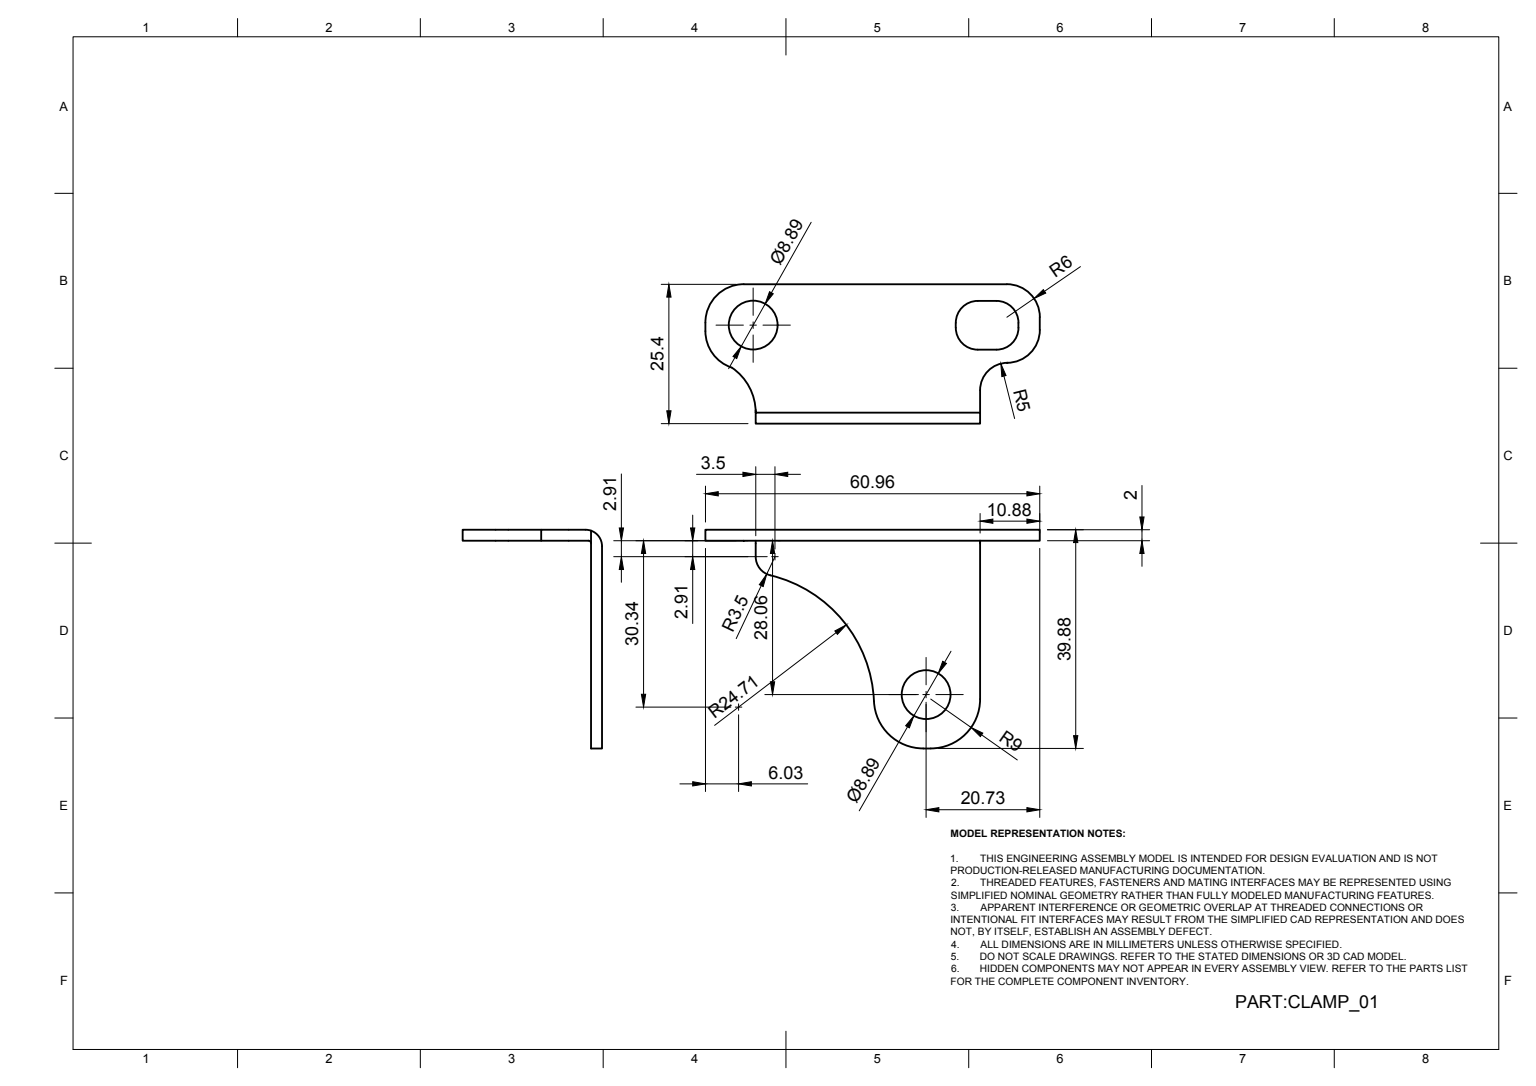
ISO-10303-21;
HEADER;
/* Generated by software containing ST-Developer
 * from STEP Tools, Inc. (www.steptools.com) 
 */

FILE_DESCRIPTION(
/* description */ (''),
/* implementation_level */ '2;1');

FILE_NAME(
/* name */ 'Clamp_01.step',
/* time_stamp */ '2026-10-04T16:49:01-07:00',
/* author */ (''),
/* organization */ (''),
/* preprocessor_version */ 'ST-DEVELOPER v20.2',
/* originating_system */ 'Autodesk Translation Framework v15.15.0.0',
/* authorisation */ '');

FILE_SCHEMA (('AUTOMOTIVE_DESIGN { 1 0 10303 214 3 1 1 }'));
ENDSEC;

DATA;
#10=MECHANICAL_DESIGN_GEOMETRIC_PRESENTATION_REPRESENTATION('',(#80),#51553);
#64=SHAPE_REPRESENTATION_RELATIONSHIP('SRR','None',#51585,#72);
#72=ADVANCED_BREP_SHAPE_REPRESENTATION('',(#89),#51545);
#80=STYLED_ITEM('',(#51634),#89);
#89=MANIFOLD_SOLID_BREP('Body1',#4259);
#98=FACE_BOUND('',#379,.T.);
#99=FACE_BOUND('',#382,.T.);
#100=FACE_BOUND('',#411,.T.);
#101=FACE_BOUND('',#412,.T.);
#102=FACE_BOUND('',#414,.T.);
#103=FACE_BOUND('',#415,.T.);
#120=PLANE('',#4363);
#121=PLANE('',#4365);
#122=PLANE('',#4371);
#123=PLANE('',#4372);
#124=PLANE('',#4383);
#125=PLANE('',#4386);
#126=PLANE('',#4390);
#127=PLANE('',#4394);
#128=PLANE('',#4398);
#129=PLANE('',#4402);
#130=PLANE('',#4415);
#131=PLANE('',#4419);
#132=PLANE('',#4423);
#133=PLANE('',#4427);
#134=PLANE('',#4428);
#135=PLANE('',#4429);
#181=FACE_OUTER_BOUND('',#376,.T.);
#182=FACE_OUTER_BOUND('',#377,.T.);
#183=FACE_OUTER_BOUND('',#378,.T.);
#184=FACE_OUTER_BOUND('',#380,.T.);
#185=FACE_OUTER_BOUND('',#381,.T.);
#186=FACE_OUTER_BOUND('',#383,.T.);
#187=FACE_OUTER_BOUND('',#384,.T.);
#188=FACE_OUTER_BOUND('',#385,.T.);
#189=FACE_OUTER_BOUND('',#386,.T.);
#190=FACE_OUTER_BOUND('',#387,.T.);
#191=FACE_OUTER_BOUND('',#388,.T.);
#192=FACE_OUTER_BOUND('',#389,.T.);
#193=FACE_OUTER_BOUND('',#390,.T.);
#194=FACE_OUTER_BOUND('',#391,.T.);
#195=FACE_OUTER_BOUND('',#392,.T.);
#196=FACE_OUTER_BOUND('',#393,.T.);
#197=FACE_OUTER_BOUND('',#394,.T.);
#198=FACE_OUTER_BOUND('',#395,.T.);
#199=FACE_OUTER_BOUND('',#396,.T.);
#200=FACE_OUTER_BOUND('',#397,.T.);
#201=FACE_OUTER_BOUND('',#398,.T.);
#202=FACE_OUTER_BOUND('',#399,.T.);
#203=FACE_OUTER_BOUND('',#400,.T.);
#204=FACE_OUTER_BOUND('',#401,.T.);
#205=FACE_OUTER_BOUND('',#402,.T.);
#206=FACE_OUTER_BOUND('',#403,.T.);
#207=FACE_OUTER_BOUND('',#404,.T.);
#208=FACE_OUTER_BOUND('',#405,.T.);
#209=FACE_OUTER_BOUND('',#406,.T.);
#210=FACE_OUTER_BOUND('',#407,.T.);
#211=FACE_OUTER_BOUND('',#408,.T.);
#212=FACE_OUTER_BOUND('',#409,.T.);
#213=FACE_OUTER_BOUND('',#410,.T.);
#214=FACE_OUTER_BOUND('',#413,.T.);
#376=EDGE_LOOP('',(#2629,#2630,#2631,#2632,#2633,#2634,#2635));
#377=EDGE_LOOP('',(#2636,#2637,#2638,#2639,#2640,#2641));
#378=EDGE_LOOP('',(#2642,#2643,#2644,#2645,#2646,#2647,#2648,#2649,#2650,
#2651));
#379=EDGE_LOOP('',(#2652));
#380=EDGE_LOOP('',(#2653,#2654,#2655,#2656));
#381=EDGE_LOOP('',(#2657,#2658,#2659,#2660,#2661,#2662,#2663,#2664));
#382=EDGE_LOOP('',(#2665));
#383=EDGE_LOOP('',(#2666,#2667,#2668,#2669));
#384=EDGE_LOOP('',(#2670,#2671,#2672,#2673));
#385=EDGE_LOOP('',(#2674,#2675,#2676,#2677));
#386=EDGE_LOOP('',(#2678,#2679,#2680,#2681));
#387=EDGE_LOOP('',(#2682,#2683,#2684,#2685));
#388=EDGE_LOOP('',(#2686,#2687,#2688,#2689));
#389=EDGE_LOOP('',(#2690,#2691,#2692,#2693));
#390=EDGE_LOOP('',(#2694,#2695,#2696,#2697,#2698,#2699,#2700));
#391=EDGE_LOOP('',(#2701,#2702,#2703,#2704));
#392=EDGE_LOOP('',(#2705,#2706,#2707,#2708));
#393=EDGE_LOOP('',(#2709,#2710,#2711,#2712));
#394=EDGE_LOOP('',(#2713,#2714,#2715,#2716));
#395=EDGE_LOOP('',(#2717,#2718,#2719,#2720));
#396=EDGE_LOOP('',(#2721,#2722,#2723,#2724));
#397=EDGE_LOOP('',(#2725,#2726,#2727,#2728));
#398=EDGE_LOOP('',(#2729,#2730,#2731,#2732));
#399=EDGE_LOOP('',(#2733,#2734,#2735,#2736));
#400=EDGE_LOOP('',(#2737,#2738,#2739,#2740));
#401=EDGE_LOOP('',(#2741,#2742,#2743,#2744,#2745));
#402=EDGE_LOOP('',(#2746,#2747,#2748,#2749));
#403=EDGE_LOOP('',(#2750,#2751,#2752,#2753));
#404=EDGE_LOOP('',(#2754,#2755,#2756,#2757));
#405=EDGE_LOOP('',(#2758,#2759,#2760,#2761));
#406=EDGE_LOOP('',(#2762,#2763,#2764,#2765));
#407=EDGE_LOOP('',(#2766,#2767,#2768,#2769));
#408=EDGE_LOOP('',(#2770,#2771,#2772,#2773));
#409=EDGE_LOOP('',(#2774,#2775,#2776,#2777));
#410=EDGE_LOOP('',(#2778,#2779,#2780,#2781,#2782,#2783,#2784,#2785,#2786,
#2787,#2788,#2789,#2790));
#411=EDGE_LOOP('',(#2791,#2792,#2793,#2794,#2795,#2796,#2797,#2798));
#412=EDGE_LOOP('',(#2799));
#413=EDGE_LOOP('',(#2800,#2801,#2802,#2803,#2804,#2805,#2806,#2807,#2808,
#2809,#2810,#2811));
#414=EDGE_LOOP('',(#2812,#2813,#2814,#2815,#2816,#2817,#2818,#2819));
#415=EDGE_LOOP('',(#2820));
#593=CIRCLE('',#4360,3.);
#594=CIRCLE('',#4361,3.);
#595=CIRCLE('',#4362,3.);
#596=CIRCLE('',#4364,0.5);
#597=CIRCLE('',#4366,3.5);
#598=CIRCLE('',#4367,24.7141941620437);
#599=CIRCLE('',#4368,9.);
#600=CIRCLE('',#4369,9.);
#601=CIRCLE('',#4370,4.445);
#602=CIRCLE('',#4373,9.);
#603=CIRCLE('',#4374,9.);
#604=CIRCLE('',#4375,24.7141941620437);
#605=CIRCLE('',#4376,3.5);
#606=CIRCLE('',#4377,4.445);
#607=CIRCLE('',#4379,0.5);
#608=CIRCLE('',#4388,4.445);
#609=CIRCLE('',#4389,4.445);
#610=CIRCLE('',#4392,3.99999999999999);
#611=CIRCLE('',#4393,3.99999999999999);
#612=CIRCLE('',#4396,4.00000000000001);
#613=CIRCLE('',#4397,4.00000000000001);
#614=CIRCLE('',#4400,4.00000000000001);
#615=CIRCLE('',#4401,4.00000000000001);
#616=CIRCLE('',#4404,4.00000000000001);
#617=CIRCLE('',#4405,4.00000000000001);
#618=CIRCLE('',#4407,6.99999999999999);
#619=CIRCLE('',#4408,6.99999999999999);
#620=CIRCLE('',#4410,9.9094315895918);
#621=CIRCLE('',#4411,9.9094315895918);
#622=CIRCLE('',#4413,5.);
#623=CIRCLE('',#4414,5.);
#624=CIRCLE('',#4417,5.99999999999999);
#625=CIRCLE('',#4418,5.99999999999999);
#626=CIRCLE('',#4421,5.99999999999999);
#627=CIRCLE('',#4422,5.99999999999999);
#628=CIRCLE('',#4425,7.);
#629=CIRCLE('',#4426,7.);
#711=LINE('',#5537,#939);
#712=LINE('',#5541,#940);
#713=LINE('',#5545,#941);
#714=LINE('',#5549,#942);
#715=LINE('',#5551,#943);
#716=LINE('',#5553,#944);
#717=LINE('',#5556,#945);
#718=LINE('',#5559,#946);
#719=LINE('',#5561,#947);
#720=LINE('',#5569,#948);
#721=LINE('',#5572,#949);
#722=LINE('',#5577,#950);
#723=LINE('',#5578,#951);
#724=LINE('',#5583,#952);
#725=LINE('',#5590,#953);
#726=LINE('',#5596,#954);
#727=LINE('',#5598,#955);
#728=LINE('',#5599,#956);
#729=LINE('',#5601,#957);
#730=LINE('',#5603,#958);
#731=LINE('',#5605,#959);
#732=LINE('',#5608,#960);
#733=LINE('',#5611,#961);
#734=LINE('',#5612,#962);
#735=LINE('',#5617,#963);
#736=LINE('',#5622,#964);
#737=LINE('',#5624,#965);
#738=LINE('',#5626,#966);
#739=LINE('',#5627,#967);
#740=LINE('',#5632,#968);
#741=LINE('',#5636,#969);
#742=LINE('',#5638,#970);
#743=LINE('',#5639,#971);
#744=LINE('',#5644,#972);
#745=LINE('',#5648,#973);
#746=LINE('',#5650,#974);
#747=LINE('',#5651,#975);
#748=LINE('',#5656,#976);
#749=LINE('',#5660,#977);
#750=LINE('',#5662,#978);
#751=LINE('',#5663,#979);
#752=LINE('',#5672,#980);
#753=LINE('',#5675,#981);
#754=LINE('',#5683,#982);
#755=LINE('',#5687,#983);
#756=LINE('',#5689,#984);
#757=LINE('',#5690,#985);
#758=LINE('',#5695,#986);
#759=LINE('',#5699,#987);
#760=LINE('',#5701,#988);
#761=LINE('',#5702,#989);
#762=LINE('',#5707,#990);
#763=LINE('',#5711,#991);
#764=LINE('',#5713,#992);
#765=LINE('',#5714,#993);
#766=LINE('',#5719,#994);
#767=LINE('',#5722,#995);
#768=LINE('',#5723,#996);
#939=VECTOR('',#4677,10.);
#940=VECTOR('',#4680,10.);
#941=VECTOR('',#4683,10.);
#942=VECTOR('',#4688,10.);
#943=VECTOR('',#4689,10.);
#944=VECTOR('',#4690,10.);
#945=VECTOR('',#4693,10.);
#946=VECTOR('',#4696,10.);
#947=VECTOR('',#4697,10.);
#948=VECTOR('',#4704,10.);
#949=VECTOR('',#4707,10.);
#950=VECTOR('',#4712,10.);
#951=VECTOR('',#4713,10.);
#952=VECTOR('',#4718,10.);
#953=VECTOR('',#4725,10.);
#954=VECTOR('',#4732,10.);
#955=VECTOR('',#4735,10.);
#956=VECTOR('',#4736,10.);
#957=VECTOR('',#4739,9.);
#958=VECTOR('',#4742,10.);
#959=VECTOR('',#4745,9.);
#960=VECTOR('',#4750,4.445);
#961=VECTOR('',#4753,10.);
#962=VECTOR('',#4754,10.);
#963=VECTOR('',#4759,4.445);
#964=VECTOR('',#4764,10.);
#965=VECTOR('',#4765,10.);
#966=VECTOR('',#4766,10.);
#967=VECTOR('',#4767,10.);
#968=VECTOR('',#4772,10.);
#969=VECTOR('',#4777,10.);
#970=VECTOR('',#4778,10.);
#971=VECTOR('',#4779,10.);
#972=VECTOR('',#4784,10.);
#973=VECTOR('',#4789,10.);
#974=VECTOR('',#4790,10.);
#975=VECTOR('',#4791,10.);
#976=VECTOR('',#4796,10.);
#977=VECTOR('',#4801,10.);
#978=VECTOR('',#4802,10.);
#979=VECTOR('',#4803,10.);
#980=VECTOR('',#4814,10.);
#981=VECTOR('',#4817,10.);
#982=VECTOR('',#4828,10.);
#983=VECTOR('',#4833,10.);
#984=VECTOR('',#4834,10.);
#985=VECTOR('',#4835,10.);
#986=VECTOR('',#4840,10.);
#987=VECTOR('',#4845,10.);
#988=VECTOR('',#4846,10.);
#989=VECTOR('',#4847,10.);
#990=VECTOR('',#4852,10.);
#991=VECTOR('',#4857,10.);
#992=VECTOR('',#4858,10.);
#993=VECTOR('',#4859,10.);
#994=VECTOR('',#4864,10.);
#995=VECTOR('',#4869,10.);
#996=VECTOR('',#4870,10.);
#1167=B_SPLINE_CURVE_WITH_KNOTS('',3,(#5532,#5533,#5534,#5535),
 .UNSPECIFIED.,.F.,.F.,(4,4),(0.459706916456031,0.558076312618392),
 .UNSPECIFIED.);
#1482=VERTEX_POINT('',#5530);
#1483=VERTEX_POINT('',#5531);
#1484=VERTEX_POINT('',#5536);
#1485=VERTEX_POINT('',#5538);
#1486=VERTEX_POINT('',#5540);
#1487=VERTEX_POINT('',#5542);
#1488=VERTEX_POINT('',#5544);
#1489=VERTEX_POINT('',#5548);
#1490=VERTEX_POINT('',#5550);
#1491=VERTEX_POINT('',#5552);
#1492=VERTEX_POINT('',#5554);
#1493=VERTEX_POINT('',#5558);
#1494=VERTEX_POINT('',#5560);
#1495=VERTEX_POINT('',#5562);
#1496=VERTEX_POINT('',#5564);
#1497=VERTEX_POINT('',#5566);
#1498=VERTEX_POINT('',#5568);
#1499=VERTEX_POINT('',#5570);
#1500=VERTEX_POINT('',#5573);
#1501=VERTEX_POINT('',#5576);
#1502=VERTEX_POINT('',#5580);
#1503=VERTEX_POINT('',#5582);
#1504=VERTEX_POINT('',#5584);
#1505=VERTEX_POINT('',#5586);
#1506=VERTEX_POINT('',#5588);
#1507=VERTEX_POINT('',#5591);
#1508=VERTEX_POINT('',#5594);
#1509=VERTEX_POINT('',#5610);
#1510=VERTEX_POINT('',#5614);
#1511=VERTEX_POINT('',#5616);
#1512=VERTEX_POINT('',#5620);
#1513=VERTEX_POINT('',#5621);
#1514=VERTEX_POINT('',#5623);
#1515=VERTEX_POINT('',#5625);
#1516=VERTEX_POINT('',#5629);
#1517=VERTEX_POINT('',#5631);
#1518=VERTEX_POINT('',#5635);
#1519=VERTEX_POINT('',#5637);
#1520=VERTEX_POINT('',#5641);
#1521=VERTEX_POINT('',#5643);
#1522=VERTEX_POINT('',#5647);
#1523=VERTEX_POINT('',#5649);
#1524=VERTEX_POINT('',#5653);
#1525=VERTEX_POINT('',#5655);
#1526=VERTEX_POINT('',#5659);
#1527=VERTEX_POINT('',#5661);
#1528=VERTEX_POINT('',#5668);
#1529=VERTEX_POINT('',#5669);
#1530=VERTEX_POINT('',#5671);
#1531=VERTEX_POINT('',#5673);
#1532=VERTEX_POINT('',#5680);
#1533=VERTEX_POINT('',#5682);
#1534=VERTEX_POINT('',#5686);
#1535=VERTEX_POINT('',#5688);
#1536=VERTEX_POINT('',#5692);
#1537=VERTEX_POINT('',#5694);
#1538=VERTEX_POINT('',#5698);
#1539=VERTEX_POINT('',#5700);
#1540=VERTEX_POINT('',#5704);
#1541=VERTEX_POINT('',#5706);
#1542=VERTEX_POINT('',#5710);
#1543=VERTEX_POINT('',#5712);
#1544=VERTEX_POINT('',#5716);
#1545=VERTEX_POINT('',#5718);
#1968=EDGE_CURVE('',#1482,#1483,#1167,.T.);
#1969=EDGE_CURVE('',#1484,#1482,#711,.T.);
#1970=EDGE_CURVE('',#1485,#1484,#593,.T.);
#1971=EDGE_CURVE('',#1486,#1485,#712,.T.);
#1972=EDGE_CURVE('',#1487,#1486,#594,.T.);
#1973=EDGE_CURVE('',#1488,#1487,#713,.T.);
#1974=EDGE_CURVE('',#1483,#1488,#595,.T.);
#1975=EDGE_CURVE('',#1489,#1484,#714,.T.);
#1976=EDGE_CURVE('',#1489,#1490,#715,.T.);
#1977=EDGE_CURVE('',#1490,#1491,#716,.T.);
#1978=EDGE_CURVE('',#1491,#1492,#596,.T.);
#1979=EDGE_CURVE('',#1485,#1492,#717,.T.);
#1980=EDGE_CURVE('',#1492,#1493,#718,.T.);
#1981=EDGE_CURVE('',#1493,#1494,#719,.T.);
#1982=EDGE_CURVE('',#1494,#1495,#597,.T.);
#1983=EDGE_CURVE('',#1496,#1495,#598,.T.);
#1984=EDGE_CURVE('',#1496,#1497,#599,.T.);
#1985=EDGE_CURVE('',#1497,#1498,#720,.T.);
#1986=EDGE_CURVE('',#1498,#1499,#600,.T.);
#1987=EDGE_CURVE('',#1486,#1499,#721,.F.);
#1988=EDGE_CURVE('',#1500,#1500,#601,.T.);
#1989=EDGE_CURVE('',#1499,#1501,#722,.T.);
#1990=EDGE_CURVE('',#1487,#1501,#723,.T.);
#1991=EDGE_CURVE('',#1501,#1502,#602,.T.);
#1992=EDGE_CURVE('',#1502,#1503,#724,.T.);
#1993=EDGE_CURVE('',#1503,#1504,#603,.T.);
#1994=EDGE_CURVE('',#1505,#1504,#604,.T.);
#1995=EDGE_CURVE('',#1505,#1506,#605,.T.);
#1996=EDGE_CURVE('',#1488,#1506,#725,.F.);
#1997=EDGE_CURVE('',#1507,#1507,#606,.T.);
#1998=EDGE_CURVE('',#1508,#1493,#607,.F.);
#1999=EDGE_CURVE('',#1508,#1491,#726,.T.);
#2000=EDGE_CURVE('',#1495,#1505,#727,.T.);
#2001=EDGE_CURVE('',#1506,#1494,#728,.T.);
#2002=EDGE_CURVE('',#1504,#1496,#729,.T.);
#2003=EDGE_CURVE('',#1502,#1498,#730,.T.);
#2004=EDGE_CURVE('',#1497,#1503,#731,.T.);
#2005=EDGE_CURVE('',#1507,#1500,#732,.T.);
#2006=EDGE_CURVE('',#1508,#1509,#733,.T.);
#2007=EDGE_CURVE('',#1483,#1509,#734,.T.);
#2008=EDGE_CURVE('',#1510,#1510,#608,.T.);
#2009=EDGE_CURVE('',#1510,#1511,#735,.T.);
#2010=EDGE_CURVE('',#1511,#1511,#609,.T.);
#2011=EDGE_CURVE('',#1512,#1513,#736,.T.);
#2012=EDGE_CURVE('',#1512,#1514,#737,.T.);
#2013=EDGE_CURVE('',#1514,#1515,#738,.T.);
#2014=EDGE_CURVE('',#1513,#1515,#739,.T.);
#2015=EDGE_CURVE('',#1516,#1512,#610,.T.);
#2016=EDGE_CURVE('',#1516,#1517,#740,.T.);
#2017=EDGE_CURVE('',#1517,#1514,#611,.T.);
#2018=EDGE_CURVE('',#1518,#1516,#741,.T.);
#2019=EDGE_CURVE('',#1518,#1519,#742,.T.);
#2020=EDGE_CURVE('',#1519,#1517,#743,.T.);
#2021=EDGE_CURVE('',#1520,#1518,#612,.T.);
#2022=EDGE_CURVE('',#1520,#1521,#744,.T.);
#2023=EDGE_CURVE('',#1521,#1519,#613,.T.);
#2024=EDGE_CURVE('',#1522,#1520,#745,.T.);
#2025=EDGE_CURVE('',#1522,#1523,#746,.T.);
#2026=EDGE_CURVE('',#1523,#1521,#747,.T.);
#2027=EDGE_CURVE('',#1524,#1522,#614,.T.);
#2028=EDGE_CURVE('',#1524,#1525,#748,.T.);
#2029=EDGE_CURVE('',#1525,#1523,#615,.T.);
#2030=EDGE_CURVE('',#1526,#1524,#749,.T.);
#2031=EDGE_CURVE('',#1526,#1527,#750,.T.);
#2032=EDGE_CURVE('',#1527,#1525,#751,.T.);
#2033=EDGE_CURVE('',#1513,#1526,#616,.T.);
#2034=EDGE_CURVE('',#1515,#1527,#617,.T.);
#2035=EDGE_CURVE('',#1528,#1529,#618,.T.);
#2036=EDGE_CURVE('',#1528,#1530,#752,.T.);
#2037=EDGE_CURVE('',#1530,#1531,#619,.T.);
#2038=EDGE_CURVE('',#1529,#1531,#753,.T.);
#2039=EDGE_CURVE('',#1509,#1530,#620,.T.);
#2040=EDGE_CURVE('',#1528,#1482,#621,.T.);
#2041=EDGE_CURVE('',#1489,#1532,#622,.T.);
#2042=EDGE_CURVE('',#1532,#1533,#754,.T.);
#2043=EDGE_CURVE('',#1533,#1490,#623,.T.);
#2044=EDGE_CURVE('',#1534,#1532,#755,.T.);
#2045=EDGE_CURVE('',#1534,#1535,#756,.T.);
#2046=EDGE_CURVE('',#1535,#1533,#757,.T.);
#2047=EDGE_CURVE('',#1536,#1534,#624,.T.);
#2048=EDGE_CURVE('',#1536,#1537,#758,.T.);
#2049=EDGE_CURVE('',#1537,#1535,#625,.T.);
#2050=EDGE_CURVE('',#1538,#1536,#759,.T.);
#2051=EDGE_CURVE('',#1538,#1539,#760,.T.);
#2052=EDGE_CURVE('',#1539,#1537,#761,.T.);
#2053=EDGE_CURVE('',#1540,#1538,#626,.T.);
#2054=EDGE_CURVE('',#1540,#1541,#762,.T.);
#2055=EDGE_CURVE('',#1541,#1539,#627,.T.);
#2056=EDGE_CURVE('',#1542,#1540,#763,.T.);
#2057=EDGE_CURVE('',#1542,#1543,#764,.T.);
#2058=EDGE_CURVE('',#1543,#1541,#765,.T.);
#2059=EDGE_CURVE('',#1544,#1542,#628,.T.);
#2060=EDGE_CURVE('',#1544,#1545,#766,.T.);
#2061=EDGE_CURVE('',#1545,#1543,#629,.T.);
#2062=EDGE_CURVE('',#1529,#1544,#767,.T.);
#2063=EDGE_CURVE('',#1531,#1545,#768,.T.);
#2629=ORIENTED_EDGE('',*,*,#1968,.F.);
#2630=ORIENTED_EDGE('',*,*,#1969,.F.);
#2631=ORIENTED_EDGE('',*,*,#1970,.F.);
#2632=ORIENTED_EDGE('',*,*,#1971,.F.);
#2633=ORIENTED_EDGE('',*,*,#1972,.F.);
#2634=ORIENTED_EDGE('',*,*,#1973,.F.);
#2635=ORIENTED_EDGE('',*,*,#1974,.F.);
#2636=ORIENTED_EDGE('',*,*,#1970,.T.);
#2637=ORIENTED_EDGE('',*,*,#1975,.F.);
#2638=ORIENTED_EDGE('',*,*,#1976,.T.);
#2639=ORIENTED_EDGE('',*,*,#1977,.T.);
#2640=ORIENTED_EDGE('',*,*,#1978,.T.);
#2641=ORIENTED_EDGE('',*,*,#1979,.F.);
#2642=ORIENTED_EDGE('',*,*,#1971,.T.);
#2643=ORIENTED_EDGE('',*,*,#1979,.T.);
#2644=ORIENTED_EDGE('',*,*,#1980,.T.);
#2645=ORIENTED_EDGE('',*,*,#1981,.T.);
#2646=ORIENTED_EDGE('',*,*,#1982,.T.);
#2647=ORIENTED_EDGE('',*,*,#1983,.F.);
#2648=ORIENTED_EDGE('',*,*,#1984,.T.);
#2649=ORIENTED_EDGE('',*,*,#1985,.T.);
#2650=ORIENTED_EDGE('',*,*,#1986,.T.);
#2651=ORIENTED_EDGE('',*,*,#1987,.F.);
#2652=ORIENTED_EDGE('',*,*,#1988,.F.);
#2653=ORIENTED_EDGE('',*,*,#1972,.T.);
#2654=ORIENTED_EDGE('',*,*,#1987,.T.);
#2655=ORIENTED_EDGE('',*,*,#1989,.T.);
#2656=ORIENTED_EDGE('',*,*,#1990,.F.);
#2657=ORIENTED_EDGE('',*,*,#1973,.T.);
#2658=ORIENTED_EDGE('',*,*,#1990,.T.);
#2659=ORIENTED_EDGE('',*,*,#1991,.T.);
#2660=ORIENTED_EDGE('',*,*,#1992,.T.);
#2661=ORIENTED_EDGE('',*,*,#1993,.T.);
#2662=ORIENTED_EDGE('',*,*,#1994,.F.);
#2663=ORIENTED_EDGE('',*,*,#1995,.T.);
#2664=ORIENTED_EDGE('',*,*,#1996,.F.);
#2665=ORIENTED_EDGE('',*,*,#1997,.F.);
#2666=ORIENTED_EDGE('',*,*,#1998,.T.);
#2667=ORIENTED_EDGE('',*,*,#1980,.F.);
#2668=ORIENTED_EDGE('',*,*,#1978,.F.);
#2669=ORIENTED_EDGE('',*,*,#1999,.F.);
#2670=ORIENTED_EDGE('',*,*,#1995,.F.);
#2671=ORIENTED_EDGE('',*,*,#2000,.F.);
#2672=ORIENTED_EDGE('',*,*,#1982,.F.);
#2673=ORIENTED_EDGE('',*,*,#2001,.F.);
#2674=ORIENTED_EDGE('',*,*,#2000,.T.);
#2675=ORIENTED_EDGE('',*,*,#1994,.T.);
#2676=ORIENTED_EDGE('',*,*,#2002,.T.);
#2677=ORIENTED_EDGE('',*,*,#1983,.T.);
#2678=ORIENTED_EDGE('',*,*,#1991,.F.);
#2679=ORIENTED_EDGE('',*,*,#1989,.F.);
#2680=ORIENTED_EDGE('',*,*,#1986,.F.);
#2681=ORIENTED_EDGE('',*,*,#2003,.F.);
#2682=ORIENTED_EDGE('',*,*,#2003,.T.);
#2683=ORIENTED_EDGE('',*,*,#1985,.F.);
#2684=ORIENTED_EDGE('',*,*,#2004,.T.);
#2685=ORIENTED_EDGE('',*,*,#1992,.F.);
#2686=ORIENTED_EDGE('',*,*,#1993,.F.);
#2687=ORIENTED_EDGE('',*,*,#2004,.F.);
#2688=ORIENTED_EDGE('',*,*,#1984,.F.);
#2689=ORIENTED_EDGE('',*,*,#2002,.F.);
#2690=ORIENTED_EDGE('',*,*,#1997,.T.);
#2691=ORIENTED_EDGE('',*,*,#2005,.T.);
#2692=ORIENTED_EDGE('',*,*,#1988,.T.);
#2693=ORIENTED_EDGE('',*,*,#2005,.F.);
#2694=ORIENTED_EDGE('',*,*,#1974,.T.);
#2695=ORIENTED_EDGE('',*,*,#1996,.T.);
#2696=ORIENTED_EDGE('',*,*,#2001,.T.);
#2697=ORIENTED_EDGE('',*,*,#1981,.F.);
#2698=ORIENTED_EDGE('',*,*,#1998,.F.);
#2699=ORIENTED_EDGE('',*,*,#2006,.T.);
#2700=ORIENTED_EDGE('',*,*,#2007,.F.);
#2701=ORIENTED_EDGE('',*,*,#2008,.T.);
#2702=ORIENTED_EDGE('',*,*,#2009,.T.);
#2703=ORIENTED_EDGE('',*,*,#2010,.F.);
#2704=ORIENTED_EDGE('',*,*,#2009,.F.);
#2705=ORIENTED_EDGE('',*,*,#2011,.F.);
#2706=ORIENTED_EDGE('',*,*,#2012,.T.);
#2707=ORIENTED_EDGE('',*,*,#2013,.T.);
#2708=ORIENTED_EDGE('',*,*,#2014,.F.);
#2709=ORIENTED_EDGE('',*,*,#2015,.F.);
#2710=ORIENTED_EDGE('',*,*,#2016,.T.);
#2711=ORIENTED_EDGE('',*,*,#2017,.T.);
#2712=ORIENTED_EDGE('',*,*,#2012,.F.);
#2713=ORIENTED_EDGE('',*,*,#2018,.F.);
#2714=ORIENTED_EDGE('',*,*,#2019,.T.);
#2715=ORIENTED_EDGE('',*,*,#2020,.T.);
#2716=ORIENTED_EDGE('',*,*,#2016,.F.);
#2717=ORIENTED_EDGE('',*,*,#2021,.F.);
#2718=ORIENTED_EDGE('',*,*,#2022,.T.);
#2719=ORIENTED_EDGE('',*,*,#2023,.T.);
#2720=ORIENTED_EDGE('',*,*,#2019,.F.);
#2721=ORIENTED_EDGE('',*,*,#2024,.F.);
#2722=ORIENTED_EDGE('',*,*,#2025,.T.);
#2723=ORIENTED_EDGE('',*,*,#2026,.T.);
#2724=ORIENTED_EDGE('',*,*,#2022,.F.);
#2725=ORIENTED_EDGE('',*,*,#2027,.F.);
#2726=ORIENTED_EDGE('',*,*,#2028,.T.);
#2727=ORIENTED_EDGE('',*,*,#2029,.T.);
#2728=ORIENTED_EDGE('',*,*,#2025,.F.);
#2729=ORIENTED_EDGE('',*,*,#2030,.F.);
#2730=ORIENTED_EDGE('',*,*,#2031,.T.);
#2731=ORIENTED_EDGE('',*,*,#2032,.T.);
#2732=ORIENTED_EDGE('',*,*,#2028,.F.);
#2733=ORIENTED_EDGE('',*,*,#2033,.F.);
#2734=ORIENTED_EDGE('',*,*,#2014,.T.);
#2735=ORIENTED_EDGE('',*,*,#2034,.T.);
#2736=ORIENTED_EDGE('',*,*,#2031,.F.);
#2737=ORIENTED_EDGE('',*,*,#2035,.F.);
#2738=ORIENTED_EDGE('',*,*,#2036,.T.);
#2739=ORIENTED_EDGE('',*,*,#2037,.T.);
#2740=ORIENTED_EDGE('',*,*,#2038,.F.);
#2741=ORIENTED_EDGE('',*,*,#1968,.T.);
#2742=ORIENTED_EDGE('',*,*,#2007,.T.);
#2743=ORIENTED_EDGE('',*,*,#2039,.T.);
#2744=ORIENTED_EDGE('',*,*,#2036,.F.);
#2745=ORIENTED_EDGE('',*,*,#2040,.T.);
#2746=ORIENTED_EDGE('',*,*,#2041,.T.);
#2747=ORIENTED_EDGE('',*,*,#2042,.T.);
#2748=ORIENTED_EDGE('',*,*,#2043,.T.);
#2749=ORIENTED_EDGE('',*,*,#1976,.F.);
#2750=ORIENTED_EDGE('',*,*,#2044,.F.);
#2751=ORIENTED_EDGE('',*,*,#2045,.T.);
#2752=ORIENTED_EDGE('',*,*,#2046,.T.);
#2753=ORIENTED_EDGE('',*,*,#2042,.F.);
#2754=ORIENTED_EDGE('',*,*,#2047,.F.);
#2755=ORIENTED_EDGE('',*,*,#2048,.T.);
#2756=ORIENTED_EDGE('',*,*,#2049,.T.);
#2757=ORIENTED_EDGE('',*,*,#2045,.F.);
#2758=ORIENTED_EDGE('',*,*,#2050,.F.);
#2759=ORIENTED_EDGE('',*,*,#2051,.T.);
#2760=ORIENTED_EDGE('',*,*,#2052,.T.);
#2761=ORIENTED_EDGE('',*,*,#2048,.F.);
#2762=ORIENTED_EDGE('',*,*,#2053,.F.);
#2763=ORIENTED_EDGE('',*,*,#2054,.T.);
#2764=ORIENTED_EDGE('',*,*,#2055,.T.);
#2765=ORIENTED_EDGE('',*,*,#2051,.F.);
#2766=ORIENTED_EDGE('',*,*,#2056,.F.);
#2767=ORIENTED_EDGE('',*,*,#2057,.T.);
#2768=ORIENTED_EDGE('',*,*,#2058,.T.);
#2769=ORIENTED_EDGE('',*,*,#2054,.F.);
#2770=ORIENTED_EDGE('',*,*,#2059,.F.);
#2771=ORIENTED_EDGE('',*,*,#2060,.T.);
#2772=ORIENTED_EDGE('',*,*,#2061,.T.);
#2773=ORIENTED_EDGE('',*,*,#2057,.F.);
#2774=ORIENTED_EDGE('',*,*,#2062,.F.);
#2775=ORIENTED_EDGE('',*,*,#2038,.T.);
#2776=ORIENTED_EDGE('',*,*,#2063,.T.);
#2777=ORIENTED_EDGE('',*,*,#2060,.F.);
#2778=ORIENTED_EDGE('',*,*,#2006,.F.);
#2779=ORIENTED_EDGE('',*,*,#1999,.T.);
#2780=ORIENTED_EDGE('',*,*,#1977,.F.);
#2781=ORIENTED_EDGE('',*,*,#2043,.F.);
#2782=ORIENTED_EDGE('',*,*,#2046,.F.);
#2783=ORIENTED_EDGE('',*,*,#2049,.F.);
#2784=ORIENTED_EDGE('',*,*,#2052,.F.);
#2785=ORIENTED_EDGE('',*,*,#2055,.F.);
#2786=ORIENTED_EDGE('',*,*,#2058,.F.);
#2787=ORIENTED_EDGE('',*,*,#2061,.F.);
#2788=ORIENTED_EDGE('',*,*,#2063,.F.);
#2789=ORIENTED_EDGE('',*,*,#2037,.F.);
#2790=ORIENTED_EDGE('',*,*,#2039,.F.);
#2791=ORIENTED_EDGE('',*,*,#2034,.F.);
#2792=ORIENTED_EDGE('',*,*,#2013,.F.);
#2793=ORIENTED_EDGE('',*,*,#2017,.F.);
#2794=ORIENTED_EDGE('',*,*,#2020,.F.);
#2795=ORIENTED_EDGE('',*,*,#2023,.F.);
#2796=ORIENTED_EDGE('',*,*,#2026,.F.);
#2797=ORIENTED_EDGE('',*,*,#2029,.F.);
#2798=ORIENTED_EDGE('',*,*,#2032,.F.);
#2799=ORIENTED_EDGE('',*,*,#2008,.F.);
#2800=ORIENTED_EDGE('',*,*,#1969,.T.);
#2801=ORIENTED_EDGE('',*,*,#2040,.F.);
#2802=ORIENTED_EDGE('',*,*,#2035,.T.);
#2803=ORIENTED_EDGE('',*,*,#2062,.T.);
#2804=ORIENTED_EDGE('',*,*,#2059,.T.);
#2805=ORIENTED_EDGE('',*,*,#2056,.T.);
#2806=ORIENTED_EDGE('',*,*,#2053,.T.);
#2807=ORIENTED_EDGE('',*,*,#2050,.T.);
#2808=ORIENTED_EDGE('',*,*,#2047,.T.);
#2809=ORIENTED_EDGE('',*,*,#2044,.T.);
#2810=ORIENTED_EDGE('',*,*,#2041,.F.);
#2811=ORIENTED_EDGE('',*,*,#1975,.T.);
#2812=ORIENTED_EDGE('',*,*,#2033,.T.);
#2813=ORIENTED_EDGE('',*,*,#2030,.T.);
#2814=ORIENTED_EDGE('',*,*,#2027,.T.);
#2815=ORIENTED_EDGE('',*,*,#2024,.T.);
#2816=ORIENTED_EDGE('',*,*,#2021,.T.);
#2817=ORIENTED_EDGE('',*,*,#2018,.T.);
#2818=ORIENTED_EDGE('',*,*,#2015,.T.);
#2819=ORIENTED_EDGE('',*,*,#2011,.T.);
#2820=ORIENTED_EDGE('',*,*,#2010,.T.);
#3951=CYLINDRICAL_SURFACE('',#4359,3.);
#3952=CYLINDRICAL_SURFACE('',#4378,0.5);
#3953=CYLINDRICAL_SURFACE('',#4380,3.5);
#3954=CYLINDRICAL_SURFACE('',#4381,24.7141941620437);
#3955=CYLINDRICAL_SURFACE('',#4382,9.);
#3956=CYLINDRICAL_SURFACE('',#4384,9.);
#3957=CYLINDRICAL_SURFACE('',#4385,4.445);
#3958=CYLINDRICAL_SURFACE('',#4387,4.445);
#3959=CYLINDRICAL_SURFACE('',#4391,3.99999999999999);
#3960=CYLINDRICAL_SURFACE('',#4395,4.00000000000001);
#3961=CYLINDRICAL_SURFACE('',#4399,4.00000000000001);
#3962=CYLINDRICAL_SURFACE('',#4403,4.00000000000001);
#3963=CYLINDRICAL_SURFACE('',#4406,6.99999999999999);
#3964=CYLINDRICAL_SURFACE('',#4409,9.9094315895918);
#3965=CYLINDRICAL_SURFACE('',#4412,5.);
#3966=CYLINDRICAL_SURFACE('',#4416,5.99999999999999);
#3967=CYLINDRICAL_SURFACE('',#4420,5.99999999999999);
#3968=CYLINDRICAL_SURFACE('',#4424,7.);
#4064=ADVANCED_FACE('',(#181),#3951,.T.);
#4065=ADVANCED_FACE('',(#182),#120,.F.);
#4066=ADVANCED_FACE('',(#183,#98),#121,.F.);
#4067=ADVANCED_FACE('',(#184),#122,.F.);
#4068=ADVANCED_FACE('',(#185,#99),#123,.F.);
#4069=ADVANCED_FACE('',(#186),#3952,.F.);
#4070=ADVANCED_FACE('',(#187),#3953,.T.);
#4071=ADVANCED_FACE('',(#188),#3954,.F.);
#4072=ADVANCED_FACE('',(#189),#3955,.T.);
#4073=ADVANCED_FACE('',(#190),#124,.F.);
#4074=ADVANCED_FACE('',(#191),#3956,.T.);
#4075=ADVANCED_FACE('',(#192),#3957,.F.);
#4076=ADVANCED_FACE('',(#193),#125,.F.);
#4077=ADVANCED_FACE('',(#194),#3958,.F.);
#4078=ADVANCED_FACE('',(#195),#126,.F.);
#4079=ADVANCED_FACE('',(#196),#3959,.F.);
#4080=ADVANCED_FACE('',(#197),#127,.F.);
#4081=ADVANCED_FACE('',(#198),#3960,.F.);
#4082=ADVANCED_FACE('',(#199),#128,.F.);
#4083=ADVANCED_FACE('',(#200),#3961,.F.);
#4084=ADVANCED_FACE('',(#201),#129,.F.);
#4085=ADVANCED_FACE('',(#202),#3962,.F.);
#4086=ADVANCED_FACE('',(#203),#3963,.T.);
#4087=ADVANCED_FACE('',(#204),#3964,.F.);
#4088=ADVANCED_FACE('',(#205),#3965,.F.);
#4089=ADVANCED_FACE('',(#206),#130,.F.);
#4090=ADVANCED_FACE('',(#207),#3966,.T.);
#4091=ADVANCED_FACE('',(#208),#131,.F.);
#4092=ADVANCED_FACE('',(#209),#3967,.T.);
#4093=ADVANCED_FACE('',(#210),#132,.F.);
#4094=ADVANCED_FACE('',(#211),#3968,.T.);
#4095=ADVANCED_FACE('',(#212),#133,.F.);
#4096=ADVANCED_FACE('',(#213,#100,#101),#134,.F.);
#4097=ADVANCED_FACE('',(#214,#102,#103),#135,.T.);
#4259=CLOSED_SHELL('',(#4064,#4065,#4066,#4067,#4068,#4069,#4070,#4071,
#4072,#4073,#4074,#4075,#4076,#4077,#4078,#4079,#4080,#4081,#4082,#4083,
#4084,#4085,#4086,#4087,#4088,#4089,#4090,#4091,#4092,#4093,#4094,#4095,
#4096,#4097));
#4358=AXIS2_PLACEMENT_3D('',#5528,#4673,#4674);
#4359=AXIS2_PLACEMENT_3D('',#5529,#4675,#4676);
#4360=AXIS2_PLACEMENT_3D('',#5539,#4678,#4679);
#4361=AXIS2_PLACEMENT_3D('',#5543,#4681,#4682);
#4362=AXIS2_PLACEMENT_3D('',#5546,#4684,#4685);
#4363=AXIS2_PLACEMENT_3D('',#5547,#4686,#4687);
#4364=AXIS2_PLACEMENT_3D('',#5555,#4691,#4692);
#4365=AXIS2_PLACEMENT_3D('',#5557,#4694,#4695);
#4366=AXIS2_PLACEMENT_3D('',#5563,#4698,#4699);
#4367=AXIS2_PLACEMENT_3D('',#5565,#4700,#4701);
#4368=AXIS2_PLACEMENT_3D('',#5567,#4702,#4703);
#4369=AXIS2_PLACEMENT_3D('',#5571,#4705,#4706);
#4370=AXIS2_PLACEMENT_3D('',#5574,#4708,#4709);
#4371=AXIS2_PLACEMENT_3D('',#5575,#4710,#4711);
#4372=AXIS2_PLACEMENT_3D('',#5579,#4714,#4715);
#4373=AXIS2_PLACEMENT_3D('',#5581,#4716,#4717);
#4374=AXIS2_PLACEMENT_3D('',#5585,#4719,#4720);
#4375=AXIS2_PLACEMENT_3D('',#5587,#4721,#4722);
#4376=AXIS2_PLACEMENT_3D('',#5589,#4723,#4724);
#4377=AXIS2_PLACEMENT_3D('',#5592,#4726,#4727);
#4378=AXIS2_PLACEMENT_3D('',#5593,#4728,#4729);
#4379=AXIS2_PLACEMENT_3D('',#5595,#4730,#4731);
#4380=AXIS2_PLACEMENT_3D('',#5597,#4733,#4734);
#4381=AXIS2_PLACEMENT_3D('',#5600,#4737,#4738);
#4382=AXIS2_PLACEMENT_3D('',#5602,#4740,#4741);
#4383=AXIS2_PLACEMENT_3D('',#5604,#4743,#4744);
#4384=AXIS2_PLACEMENT_3D('',#5606,#4746,#4747);
#4385=AXIS2_PLACEMENT_3D('',#5607,#4748,#4749);
#4386=AXIS2_PLACEMENT_3D('',#5609,#4751,#4752);
#4387=AXIS2_PLACEMENT_3D('',#5613,#4755,#4756);
#4388=AXIS2_PLACEMENT_3D('',#5615,#4757,#4758);
#4389=AXIS2_PLACEMENT_3D('',#5618,#4760,#4761);
#4390=AXIS2_PLACEMENT_3D('',#5619,#4762,#4763);
#4391=AXIS2_PLACEMENT_3D('',#5628,#4768,#4769);
#4392=AXIS2_PLACEMENT_3D('',#5630,#4770,#4771);
#4393=AXIS2_PLACEMENT_3D('',#5633,#4773,#4774);
#4394=AXIS2_PLACEMENT_3D('',#5634,#4775,#4776);
#4395=AXIS2_PLACEMENT_3D('',#5640,#4780,#4781);
#4396=AXIS2_PLACEMENT_3D('',#5642,#4782,#4783);
#4397=AXIS2_PLACEMENT_3D('',#5645,#4785,#4786);
#4398=AXIS2_PLACEMENT_3D('',#5646,#4787,#4788);
#4399=AXIS2_PLACEMENT_3D('',#5652,#4792,#4793);
#4400=AXIS2_PLACEMENT_3D('',#5654,#4794,#4795);
#4401=AXIS2_PLACEMENT_3D('',#5657,#4797,#4798);
#4402=AXIS2_PLACEMENT_3D('',#5658,#4799,#4800);
#4403=AXIS2_PLACEMENT_3D('',#5664,#4804,#4805);
#4404=AXIS2_PLACEMENT_3D('',#5665,#4806,#4807);
#4405=AXIS2_PLACEMENT_3D('',#5666,#4808,#4809);
#4406=AXIS2_PLACEMENT_3D('',#5667,#4810,#4811);
#4407=AXIS2_PLACEMENT_3D('',#5670,#4812,#4813);
#4408=AXIS2_PLACEMENT_3D('',#5674,#4815,#4816);
#4409=AXIS2_PLACEMENT_3D('',#5676,#4818,#4819);
#4410=AXIS2_PLACEMENT_3D('',#5677,#4820,#4821);
#4411=AXIS2_PLACEMENT_3D('',#5678,#4822,#4823);
#4412=AXIS2_PLACEMENT_3D('',#5679,#4824,#4825);
#4413=AXIS2_PLACEMENT_3D('',#5681,#4826,#4827);
#4414=AXIS2_PLACEMENT_3D('',#5684,#4829,#4830);
#4415=AXIS2_PLACEMENT_3D('',#5685,#4831,#4832);
#4416=AXIS2_PLACEMENT_3D('',#5691,#4836,#4837);
#4417=AXIS2_PLACEMENT_3D('',#5693,#4838,#4839);
#4418=AXIS2_PLACEMENT_3D('',#5696,#4841,#4842);
#4419=AXIS2_PLACEMENT_3D('',#5697,#4843,#4844);
#4420=AXIS2_PLACEMENT_3D('',#5703,#4848,#4849);
#4421=AXIS2_PLACEMENT_3D('',#5705,#4850,#4851);
#4422=AXIS2_PLACEMENT_3D('',#5708,#4853,#4854);
#4423=AXIS2_PLACEMENT_3D('',#5709,#4855,#4856);
#4424=AXIS2_PLACEMENT_3D('',#5715,#4860,#4861);
#4425=AXIS2_PLACEMENT_3D('',#5717,#4862,#4863);
#4426=AXIS2_PLACEMENT_3D('',#5720,#4865,#4866);
#4427=AXIS2_PLACEMENT_3D('',#5721,#4867,#4868);
#4428=AXIS2_PLACEMENT_3D('',#5724,#4871,#4872);
#4429=AXIS2_PLACEMENT_3D('',#5725,#4873,#4874);
#4673=DIRECTION('axis',(0.,0.,1.));
#4674=DIRECTION('refdir',(1.,0.,0.));
#4675=DIRECTION('center_axis',(-1.,-1.22464679914735E-16,2.71926214689378E-32));
#4676=DIRECTION('ref_axis',(-8.65956056235492E-17,0.707106781186548,-0.707106781186547));
#4677=DIRECTION('',(-1.,-1.22464679914735E-16,2.71926214689378E-32));
#4678=DIRECTION('center_axis',(1.,1.22464679914735E-16,-2.71926214689378E-32));
#4679=DIRECTION('ref_axis',(-8.65956056235492E-17,0.707106781186548,-0.707106781186547));
#4680=DIRECTION('',(-1.,-1.22464679914735E-16,2.71926214689378E-32));
#4681=DIRECTION('center_axis',(1.,1.22464679914734E-16,-4.44089209850062E-15));
#4682=DIRECTION('ref_axis',(-3.22678052299109E-15,0.707106781186548,-0.707106781186547));
#4683=DIRECTION('',(1.,1.22464679914735E-16,-2.71926214689378E-32));
#4684=DIRECTION('center_axis',(-1.,-1.22464679914735E-16,6.9563080245457E-32));
#4685=DIRECTION('ref_axis',(-8.65956056235492E-17,0.707106781186548,-0.707106781186547));
#4686=DIRECTION('center_axis',(-1.,-1.22464679914735E-16,2.71926214689378E-32));
#4687=DIRECTION('ref_axis',(-8.75811540203011E-47,-2.22044604925031E-16,
-1.));
#4688=DIRECTION('',(0.,-2.22044604925031E-16,-1.));
#4689=DIRECTION('',(1.22464679914735E-16,-1.,2.22044604925031E-16));
#4690=DIRECTION('',(0.,-2.22044604925031E-16,-1.));
#4691=DIRECTION('center_axis',(-1.,-1.22464679914735E-16,2.71926214689378E-32));
#4692=DIRECTION('ref_axis',(-8.65956056235493E-17,0.707106781186549,-0.707106781186547));
#4693=DIRECTION('',(1.22464679914735E-16,-1.,2.22044604925031E-16));
#4694=DIRECTION('center_axis',(0.,-2.22044604925031E-16,-1.));
#4695=DIRECTION('ref_axis',(1.,1.22464679914735E-16,-2.71926214689377E-32));
#4696=DIRECTION('',(-1.,-1.22464679914735E-16,2.71926214689378E-32));
#4697=DIRECTION('',(1.22464679914735E-16,-1.,2.22044604925031E-16));
#4698=DIRECTION('center_axis',(0.,2.22044604925031E-16,1.));
#4699=DIRECTION('ref_axis',(-0.785839144811216,-0.61843094883938,1.37319255708452E-16));
#4700=DIRECTION('center_axis',(0.,2.22044604925031E-16,1.));
#4701=DIRECTION('ref_axis',(0.126759996397889,0.991933416774134,-2.20253463639549E-16));
#4702=DIRECTION('center_axis',(0.,2.22044604925031E-16,1.));
#4703=DIRECTION('ref_axis',(-1.22464679914735E-16,1.,-2.22044604925031E-16));
#4704=DIRECTION('',(1.,1.22464679914735E-16,-2.71926214689378E-32));
#4705=DIRECTION('center_axis',(0.,2.22044604925031E-16,1.));
#4706=DIRECTION('ref_axis',(0.707106781186548,-0.707106781186547,1.57009245868377E-16));
#4707=DIRECTION('',(-1.22464679914735E-16,1.,-2.22044604925031E-16));
#4708=DIRECTION('center_axis',(0.,2.22044604925031E-16,1.));
#4709=DIRECTION('ref_axis',(1.,1.22464679914735E-16,-2.71926214689377E-32));
#4710=DIRECTION('center_axis',(-1.,-1.22464679914734E-16,4.44089209850062E-15));
#4711=DIRECTION('ref_axis',(-4.44089209850062E-15,-2.22044604925032E-16,
-1.));
#4712=DIRECTION('',(-4.44089209850062E-15,-2.22044604925032E-16,-1.));
#4713=DIRECTION('',(1.22464679914735E-16,-1.,2.22044604925031E-16));
#4714=DIRECTION('center_axis',(0.,2.22044604925031E-16,1.));
#4715=DIRECTION('ref_axis',(-1.,-1.22464679914735E-16,2.71926214689377E-32));
#4716=DIRECTION('center_axis',(0.,-2.22044604925031E-16,-1.));
#4717=DIRECTION('ref_axis',(0.707106781186548,-0.707106781186547,1.57009245868377E-16));
#4718=DIRECTION('',(-1.,-1.22464679914735E-16,2.71926214689378E-32));
#4719=DIRECTION('center_axis',(0.,-2.22044604925031E-16,-1.));
#4720=DIRECTION('ref_axis',(-1.22464679914735E-16,1.,-2.22044604925031E-16));
#4721=DIRECTION('center_axis',(0.,-2.22044604925031E-16,-1.));
#4722=DIRECTION('ref_axis',(0.126759996397889,0.991933416774134,-2.20253463639549E-16));
#4723=DIRECTION('center_axis',(0.,-2.22044604925031E-16,-1.));
#4724=DIRECTION('ref_axis',(-0.785839144811216,-0.61843094883938,1.37319255708452E-16));
#4725=DIRECTION('',(-1.22464679914735E-16,1.,-2.22044604925031E-16));
#4726=DIRECTION('center_axis',(0.,-2.22044604925031E-16,-1.));
#4727=DIRECTION('ref_axis',(1.,1.22464679914735E-16,-2.71926214689377E-32));
#4728=DIRECTION('center_axis',(1.,1.22464679914735E-16,-2.71926214689378E-32));
#4729=DIRECTION('ref_axis',(-8.65956056235493E-17,0.707106781186549,-0.707106781186547));
#4730=DIRECTION('center_axis',(1.,1.22464679914735E-16,-6.9563080245457E-32));
#4731=DIRECTION('ref_axis',(-8.65956056235493E-17,0.707106781186549,-0.707106781186547));
#4732=DIRECTION('',(1.,1.22464679914735E-16,-2.71926214689378E-32));
#4733=DIRECTION('center_axis',(0.,2.22044604925031E-16,1.));
#4734=DIRECTION('ref_axis',(-0.785839144811216,-0.61843094883938,1.37319255708452E-16));
#4735=DIRECTION('',(0.,-2.22044604925031E-16,-1.));
#4736=DIRECTION('',(4.23704587765192E-32,2.22044604925031E-16,1.));
#4737=DIRECTION('center_axis',(0.,2.22044604925031E-16,1.));
#4738=DIRECTION('ref_axis',(0.126759996397889,0.991933416774134,-2.20253463639549E-16));
#4739=DIRECTION('',(0.,2.22044604925031E-16,1.));
#4740=DIRECTION('center_axis',(4.44089209850062E-15,2.22044604925032E-16,
1.));
#4741=DIRECTION('ref_axis',(0.707106781186548,-0.707106781186547,-2.98317567149917E-15));
#4742=DIRECTION('',(4.44089209850062E-15,2.22044604925032E-16,1.));
#4743=DIRECTION('center_axis',(-1.22464679914735E-16,1.,-2.22044604925031E-16));
#4744=DIRECTION('ref_axis',(1.,1.22464679914735E-16,-2.71926214689378E-32));
#4745=DIRECTION('',(0.,-2.22044604925031E-16,-1.));
#4746=DIRECTION('center_axis',(0.,-2.22044604925031E-16,-1.));
#4747=DIRECTION('ref_axis',(-1.22464679914735E-16,1.,-2.22044604925031E-16));
#4748=DIRECTION('center_axis',(0.,2.22044604925031E-16,1.));
#4749=DIRECTION('ref_axis',(1.,1.22464679914735E-16,-2.71926214689377E-32));
#4750=DIRECTION('',(0.,2.22044604925031E-16,1.));
#4751=DIRECTION('center_axis',(1.,1.22464679914735E-16,-6.9563080245457E-32));
#4752=DIRECTION('ref_axis',(4.23704587765193E-32,2.22044604925031E-16,1.));
#4753=DIRECTION('',(-4.23704587765192E-32,-2.22044604925031E-16,-1.));
#4754=DIRECTION('',(1.22464679914735E-16,-1.,2.22044604925031E-16));
#4755=DIRECTION('center_axis',(-1.22464679914735E-16,1.,-2.22044604925031E-16));
#4756=DIRECTION('ref_axis',(1.,1.22464679914735E-16,-2.71926214689378E-32));
#4757=DIRECTION('center_axis',(1.22464679914735E-16,-1.,2.22044604925031E-16));
#4758=DIRECTION('ref_axis',(1.,1.22464679914735E-16,-2.71926214689378E-32));
#4759=DIRECTION('',(-1.22464679914735E-16,1.,-2.22044604925031E-16));
#4760=DIRECTION('center_axis',(1.22464679914735E-16,-1.,2.22044604925031E-16));
#4761=DIRECTION('ref_axis',(1.,1.22464679914735E-16,-2.71926214689378E-32));
#4762=DIRECTION('center_axis',(1.,1.22464679914735E-16,-2.71926214689378E-32));
#4763=DIRECTION('ref_axis',(8.75811540203011E-47,2.22044604925031E-16,1.));
#4764=DIRECTION('',(0.,2.22044604925031E-16,1.));
#4765=DIRECTION('',(1.22464679914735E-16,-1.,2.22044604925031E-16));
#4766=DIRECTION('',(0.,2.22044604925031E-16,1.));
#4767=DIRECTION('',(1.22464679914735E-16,-1.,2.22044604925031E-16));
#4768=DIRECTION('center_axis',(-1.22464679914735E-16,1.,-2.22044604925031E-16));
#4769=DIRECTION('ref_axis',(1.,1.22464679914735E-16,2.77555756156289E-16));
#4770=DIRECTION('center_axis',(1.22464679914735E-16,-1.,2.22044604925031E-16));
#4771=DIRECTION('ref_axis',(1.,1.22464679914735E-16,2.77555756156289E-16));
#4772=DIRECTION('',(1.22464679914735E-16,-1.,2.22044604925031E-16));
#4773=DIRECTION('center_axis',(1.22464679914735E-16,-1.,2.22044604925031E-16));
#4774=DIRECTION('ref_axis',(1.,1.22464679914735E-16,2.77555756156289E-16));
#4775=DIRECTION('center_axis',(1.29472072842584E-15,-2.22044604925031E-16,
-1.));
#4776=DIRECTION('ref_axis',(1.,1.22464679914736E-16,1.29472072842584E-15));
#4777=DIRECTION('',(1.,1.22464679914736E-16,1.29472072842584E-15));
#4778=DIRECTION('',(1.22464679914735E-16,-1.,2.22044604925031E-16));
#4779=DIRECTION('',(1.,1.22464679914736E-16,1.29472072842584E-15));
#4780=DIRECTION('center_axis',(-1.22464679914735E-16,1.,-2.22044604925031E-16));
#4781=DIRECTION('ref_axis',(2.08890553820447E-48,-2.22044604925031E-16,
-1.));
#4782=DIRECTION('center_axis',(1.22464679914735E-16,-1.,2.22044604925031E-16));
#4783=DIRECTION('ref_axis',(2.08890553820447E-48,-2.22044604925031E-16,
-1.));
#4784=DIRECTION('',(1.22464679914735E-16,-1.,2.22044604925031E-16));
#4785=DIRECTION('center_axis',(1.22464679914735E-16,-1.,2.22044604925031E-16));
#4786=DIRECTION('ref_axis',(2.08890553820447E-48,-2.22044604925031E-16,
-1.));
#4787=DIRECTION('center_axis',(-1.,-1.22464679914735E-16,2.71926214689378E-32));
#4788=DIRECTION('ref_axis',(-8.75811540203011E-47,-2.22044604925031E-16,
-1.));
#4789=DIRECTION('',(0.,-2.22044604925031E-16,-1.));
#4790=DIRECTION('',(1.22464679914735E-16,-1.,2.22044604925031E-16));
#4791=DIRECTION('',(0.,-2.22044604925031E-16,-1.));
#4792=DIRECTION('center_axis',(-1.22464679914735E-16,1.,-2.22044604925031E-16));
#4793=DIRECTION('ref_axis',(-1.,-1.22464679914735E-16,1.66533453693773E-15));
#4794=DIRECTION('center_axis',(1.22464679914735E-16,-1.,2.22044604925031E-16));
#4795=DIRECTION('ref_axis',(-1.,-1.22464679914735E-16,1.66533453693773E-15));
#4796=DIRECTION('',(1.22464679914735E-16,-1.,2.22044604925031E-16));
#4797=DIRECTION('center_axis',(1.22464679914735E-16,-1.,2.22044604925031E-16));
#4798=DIRECTION('ref_axis',(-1.,-1.22464679914735E-16,1.66533453693773E-15));
#4799=DIRECTION('center_axis',(8.09200455266149E-16,2.22044604925031E-16,
1.));
#4800=DIRECTION('ref_axis',(-1.,-1.22464679914735E-16,8.09200455266149E-16));
#4801=DIRECTION('',(-1.,-1.22464679914735E-16,8.09200455266149E-16));
#4802=DIRECTION('',(1.22464679914735E-16,-1.,2.22044604925031E-16));
#4803=DIRECTION('',(-1.,-1.22464679914735E-16,8.09200455266149E-16));
#4804=DIRECTION('center_axis',(-1.22464679914735E-16,1.,-2.22044604925031E-16));
#4805=DIRECTION('ref_axis',(2.22044604925031E-15,2.22044604925031E-16,1.));
#4806=DIRECTION('center_axis',(1.22464679914735E-16,-1.,2.22044604925031E-16));
#4807=DIRECTION('ref_axis',(2.22044604925031E-15,2.22044604925031E-16,1.));
#4808=DIRECTION('center_axis',(1.22464679914735E-16,-1.,2.22044604925031E-16));
#4809=DIRECTION('ref_axis',(2.22044604925031E-15,2.22044604925031E-16,1.));
#4810=DIRECTION('center_axis',(-1.22464679914735E-16,1.,-2.22044604925031E-16));
#4811=DIRECTION('ref_axis',(1.58603289232165E-16,-2.22044604925031E-16,
-1.));
#4812=DIRECTION('center_axis',(-1.22464679914735E-16,1.,-2.22044604925031E-16));
#4813=DIRECTION('ref_axis',(1.58603289232165E-16,-2.22044604925031E-16,
-1.));
#4814=DIRECTION('',(1.22464679914735E-16,-1.,2.22044604925031E-16));
#4815=DIRECTION('center_axis',(-1.22464679914735E-16,1.,-2.22044604925031E-16));
#4816=DIRECTION('ref_axis',(1.58603289232165E-16,-2.22044604925031E-16,
-1.));
#4817=DIRECTION('',(1.22464679914735E-16,-1.,2.22044604925031E-16));
#4818=DIRECTION('center_axis',(-1.22464679914735E-16,1.,-2.22044604925031E-16));
#4819=DIRECTION('ref_axis',(0.559779357098146,2.52548619278702E-16,0.828641702647644));
#4820=DIRECTION('center_axis',(1.22464679914735E-16,-1.,2.22044604925031E-16));
#4821=DIRECTION('ref_axis',(0.559779357098146,2.52548619278702E-16,0.828641702647644));
#4822=DIRECTION('center_axis',(-1.22464679914735E-16,1.,-2.22044604925031E-16));
#4823=DIRECTION('ref_axis',(0.559779357098146,2.52548619278702E-16,0.828641702647644));
#4824=DIRECTION('center_axis',(-1.22464679914735E-16,1.,-2.22044604925031E-16));
#4825=DIRECTION('ref_axis',(-1.,-1.22464679914735E-16,2.71926214689378E-32));
#4826=DIRECTION('center_axis',(-1.22464679914735E-16,1.,-2.22044604925031E-16));
#4827=DIRECTION('ref_axis',(-1.,-1.22464679914735E-16,2.71926214689378E-32));
#4828=DIRECTION('',(1.22464679914735E-16,-1.,2.22044604925031E-16));
#4829=DIRECTION('center_axis',(1.22464679914735E-16,-1.,2.22044604925031E-16));
#4830=DIRECTION('ref_axis',(-1.,-1.22464679914735E-16,2.71926214689378E-32));
#4831=DIRECTION('center_axis',(-1.90049007730895E-14,-2.22044604925034E-16,
-1.));
#4832=DIRECTION('ref_axis',(1.,1.22464679914731E-16,-1.90049007730895E-14));
#4833=DIRECTION('',(1.,1.22464679914731E-16,-1.90049007730895E-14));
#4834=DIRECTION('',(1.22464679914735E-16,-1.,2.22044604925031E-16));
#4835=DIRECTION('',(1.,1.22464679914731E-16,-1.90049007730895E-14));
#4836=DIRECTION('center_axis',(-1.22464679914735E-16,1.,-2.22044604925031E-16));
#4837=DIRECTION('ref_axis',(1.,1.22464679914735E-16,-2.71926214689378E-32));
#4838=DIRECTION('center_axis',(-1.22464679914735E-16,1.,-2.22044604925031E-16));
#4839=DIRECTION('ref_axis',(1.,1.22464679914735E-16,-2.71926214689378E-32));
#4840=DIRECTION('',(1.22464679914735E-16,-1.,2.22044604925031E-16));
#4841=DIRECTION('center_axis',(-1.22464679914735E-16,1.,-2.22044604925031E-16));
#4842=DIRECTION('ref_axis',(1.,1.22464679914735E-16,-2.71926214689378E-32));
#4843=DIRECTION('center_axis',(-1.,-1.22464679914735E-16,2.71926214689378E-32));
#4844=DIRECTION('ref_axis',(-8.75811540203011E-47,-2.22044604925031E-16,
-1.));
#4845=DIRECTION('',(0.,-2.22044604925031E-16,-1.));
#4846=DIRECTION('',(1.22464679914735E-16,-1.,2.22044604925031E-16));
#4847=DIRECTION('',(0.,-2.22044604925031E-16,-1.));
#4848=DIRECTION('center_axis',(-1.22464679914735E-16,1.,-2.22044604925031E-16));
#4849=DIRECTION('ref_axis',(-1.48029736616688E-15,2.22044604925031E-16,
1.));
#4850=DIRECTION('center_axis',(-1.22464679914735E-16,1.,-2.22044604925031E-16));
#4851=DIRECTION('ref_axis',(-1.48029736616688E-15,2.22044604925031E-16,
1.));
#4852=DIRECTION('',(1.22464679914735E-16,-1.,2.22044604925031E-16));
#4853=DIRECTION('center_axis',(-1.22464679914735E-16,1.,-2.22044604925031E-16));
#4854=DIRECTION('ref_axis',(-1.48029736616688E-15,2.22044604925031E-16,
1.));
#4855=DIRECTION('center_axis',(0.,-2.22044604925031E-16,-1.));
#4856=DIRECTION('ref_axis',(1.,1.22464679914735E-16,-2.71926214689377E-32));
#4857=DIRECTION('',(1.,1.22464679914735E-16,-2.71926214689378E-32));
#4858=DIRECTION('',(1.22464679914735E-16,-1.,2.22044604925031E-16));
#4859=DIRECTION('',(1.,1.22464679914735E-16,-2.71926214689378E-32));
#4860=DIRECTION('center_axis',(-1.22464679914735E-16,1.,-2.22044604925031E-16));
#4861=DIRECTION('ref_axis',(-1.,-1.22464679914735E-16,2.71926214689378E-32));
#4862=DIRECTION('center_axis',(-1.22464679914735E-16,1.,-2.22044604925031E-16));
#4863=DIRECTION('ref_axis',(-1.,-1.22464679914735E-16,2.71926214689378E-32));
#4864=DIRECTION('',(1.22464679914735E-16,-1.,2.22044604925031E-16));
#4865=DIRECTION('center_axis',(-1.22464679914735E-16,1.,-2.22044604925031E-16));
#4866=DIRECTION('ref_axis',(-1.,-1.22464679914735E-16,2.71926214689378E-32));
#4867=DIRECTION('center_axis',(1.,1.22464679914735E-16,-1.44006500428221E-15));
#4868=DIRECTION('ref_axis',(1.44006500428221E-15,2.22044604925031E-16,1.));
#4869=DIRECTION('',(1.44006500428221E-15,2.22044604925031E-16,1.));
#4870=DIRECTION('',(1.44006500428221E-15,2.22044604925031E-16,1.));
#4871=DIRECTION('center_axis',(-1.22464679914735E-16,1.,-2.22044604925031E-16));
#4872=DIRECTION('ref_axis',(1.,1.22464679914735E-16,-2.71926214689378E-32));
#4873=DIRECTION('center_axis',(-1.22464679914735E-16,1.,-2.22044604925031E-16));
#4874=DIRECTION('ref_axis',(1.,1.22464679914735E-16,-2.71926214689378E-32));
#5528=CARTESIAN_POINT('',(0.,0.,0.));
#5529=CARTESIAN_POINT('Origin',(9.94695118785088,27.0570908269895,11.9861373773513));
#5530=CARTESIAN_POINT('',(-26.6569870402034,30.0570908269895,11.9861373773513));
#5531=CARTESIAN_POINT('',(-26.6064009422907,29.8855179517357,10.9861373773513));
#5532=CARTESIAN_POINT('Ctrl Pts',(-26.6569870402035,30.0570908269895,11.9861373773513));
#5533=CARTESIAN_POINT('Ctrl Pts',(-26.6238975552776,30.0570908269895,11.6599132580678));
#5534=CARTESIAN_POINT('Ctrl Pts',(-26.6064009422907,30.0012679867952,11.3135279162041));
#5535=CARTESIAN_POINT('Ctrl Pts',(-26.6064009422907,29.8855179517357,10.9861373773513));
#5536=CARTESIAN_POINT('',(14.3037866333901,30.0570908269895,11.9861373773513));
#5537=CARTESIAN_POINT('',(9.94695118785088,30.0570908269895,11.9861373773513));
#5538=CARTESIAN_POINT('',(14.3037866333901,29.8855179517357,10.9861373773513));
#5539=CARTESIAN_POINT('Origin',(14.3037866333901,27.0570908269895,11.9861373773513));
#5540=CARTESIAN_POINT('',(14.3039511878509,29.8855179517357,10.9861373773513));
#5541=CARTESIAN_POINT('',(9.94695118785088,29.8855179517357,10.9861373773513));
#5542=CARTESIAN_POINT('',(14.3039511878509,27.0570908269895,8.98613737735134));
#5543=CARTESIAN_POINT('Origin',(14.3039511878509,27.0570908269895,11.9861373773513));
#5544=CARTESIAN_POINT('',(-26.6060488121491,27.0570908269895,8.98613737735134));
#5545=CARTESIAN_POINT('',(9.94695118785088,27.0570908269895,8.98613737735134));
#5546=CARTESIAN_POINT('Origin',(-26.6060488121491,27.0570908269895,11.9861373773513));
#5547=CARTESIAN_POINT('Origin',(14.3037866333901,30.0570908269895,15.0708658676184));
#5548=CARTESIAN_POINT('',(14.3037866333901,30.0570908269895,15.0708658676184));
#5549=CARTESIAN_POINT('',(14.3037866333901,30.0570908269895,15.0708658676184));
#5550=CARTESIAN_POINT('',(14.3037866333901,28.0570908269895,15.0708658676184));
#5551=CARTESIAN_POINT('',(14.3037866333901,30.0570908269895,15.0708658676184));
#5552=CARTESIAN_POINT('',(14.3037866333901,28.0570908269895,11.4861373773513));
#5553=CARTESIAN_POINT('',(14.3037866333901,28.0570908269895,15.0708658676184));
#5554=CARTESIAN_POINT('',(14.3037866333901,27.5570908269895,10.9861373773513));
#5555=CARTESIAN_POINT('Origin',(14.3037866333901,27.5570908269895,11.4861373773513));
#5556=CARTESIAN_POINT('',(14.3037866333901,30.0570908269895,10.9861373773513));
#5557=CARTESIAN_POINT('Origin',(-35.7730488121491,30.0570908269895,10.9861373773513));
#5558=CARTESIAN_POINT('',(-26.6060488121491,27.5570908269895,10.9861373773513));
#5559=CARTESIAN_POINT('',(-20.5330488121491,27.5570908269895,10.9861373773513));
#5560=CARTESIAN_POINT('',(-26.6060488121491,25.1429698676036,10.9861373773513));
#5561=CARTESIAN_POINT('',(-26.6060488121491,30.0570908269895,10.9861373773513));
#5562=CARTESIAN_POINT('',(-23.9288509427725,21.7410591318785,10.9861373773513));
#5563=CARTESIAN_POINT('Origin',(-23.1060488121491,25.1429698676036,10.9861373773513));
#5564=CARTESIAN_POINT('',(-5.04779768493513,-1.21054870903725,10.9861373773513));
#5565=CARTESIAN_POINT('Origin',(-29.7388199751065,-2.28050728087887,10.9861373773513));
#5566=CARTESIAN_POINT('',(3.94376397208333,-9.82090917301047,10.9861373773513));
#5567=CARTESIAN_POINT('Origin',(3.94376397208333,-0.820909173010468,10.9861373773513));
#5568=CARTESIAN_POINT('',(5.30395118785094,-9.82090917301047,10.9861373773513));
#5569=CARTESIAN_POINT('',(25.1869511878509,-9.82090917301046,10.9861373773513));
#5570=CARTESIAN_POINT('',(14.3039511878509,-0.820909173010467,10.9861373773513));
#5571=CARTESIAN_POINT('Origin',(5.30395118785094,-0.820909173010468,10.9861373773512));
#5572=CARTESIAN_POINT('',(14.3039511878509,30.0570908269895,10.9861373773513));
#5573=CARTESIAN_POINT('',(0.0114691062182715,3.00528005601026E-15,10.9861373773513));
#5574=CARTESIAN_POINT('Origin',(4.45646910621825,3.54963555823125E-15,10.9861373773513));
#5575=CARTESIAN_POINT('Origin',(14.3039511878509,30.0570908269895,10.9861373773514));
#5576=CARTESIAN_POINT('',(14.3039511878509,-0.820909173010467,8.98613737735134));
#5577=CARTESIAN_POINT('',(14.3039511878509,-0.820909173010467,10.4861373773513));
#5578=CARTESIAN_POINT('',(14.3039511878509,30.0570908269895,8.98613737735134));
#5579=CARTESIAN_POINT('Origin',(25.1869511878509,30.0570908269895,8.98613737735134));
#5580=CARTESIAN_POINT('',(5.30395118785094,-9.82090917301047,8.98613737735135));
#5581=CARTESIAN_POINT('Origin',(5.30395118785094,-0.820909173010468,8.98613737735143));
#5582=CARTESIAN_POINT('',(3.94376397208333,-9.82090917301047,8.98613737735135));
#5583=CARTESIAN_POINT('',(-35.7730488121491,-9.82090917301047,8.98613737735135));
#5584=CARTESIAN_POINT('',(-5.04779768493513,-1.21054870903725,8.98613737735134));
#5585=CARTESIAN_POINT('Origin',(3.94376397208333,-0.820909173010468,8.98613737735134));
#5586=CARTESIAN_POINT('',(-23.9288509427725,21.7410591318785,8.98613737735134));
#5587=CARTESIAN_POINT('Origin',(-29.7388199751065,-2.28050728087887,8.98613737735134));
#5588=CARTESIAN_POINT('',(-26.6060488121491,25.1429698676036,8.98613737735134));
#5589=CARTESIAN_POINT('Origin',(-23.1060488121491,25.1429698676036,8.98613737735134));
#5590=CARTESIAN_POINT('',(-26.6060488121491,30.0570908269895,8.98613737735134));
#5591=CARTESIAN_POINT('',(0.0114691062182715,2.5611908461602E-15,8.98613737735134));
#5592=CARTESIAN_POINT('Origin',(4.45646910621825,3.10554634838119E-15,8.98613737735134));
#5593=CARTESIAN_POINT('Origin',(-20.5330488121491,27.5570908269895,11.4861373773513));
#5594=CARTESIAN_POINT('',(-26.6060488121491,28.0570908269895,11.4861373773513));
#5595=CARTESIAN_POINT('Origin',(-26.6060488121491,27.5570908269895,11.4861373773513));
#5596=CARTESIAN_POINT('',(-20.5330488121491,28.0570908269895,11.4861373773513));
#5597=CARTESIAN_POINT('Origin',(-23.1060488121491,25.1429698676036,10.9861373773513));
#5598=CARTESIAN_POINT('',(-23.9288509427725,21.7410591318785,10.9861373773513));
#5599=CARTESIAN_POINT('',(-26.6060488121491,25.1429698676036,10.9861373773513));
#5600=CARTESIAN_POINT('Origin',(-29.7388199751065,-2.28050728087887,10.9861373773513));
#5601=CARTESIAN_POINT('',(-5.04779768493513,-1.21054870903725,10.9861373773513));
#5602=CARTESIAN_POINT('Origin',(5.30395118785094,-0.820909173010468,10.4861373773514));
#5603=CARTESIAN_POINT('',(5.30395118785094,-9.82090917301047,10.4861373773514));
#5604=CARTESIAN_POINT('Origin',(-5.29304881214905,-9.82090917301047,9.98613737735135));
#5605=CARTESIAN_POINT('',(3.94376397208333,-9.82090917301047,10.9861373773513));
#5606=CARTESIAN_POINT('Origin',(3.94376397208333,-0.820909173010468,10.9861373773513));
#5607=CARTESIAN_POINT('Origin',(4.45646910621825,3.54963555823125E-15,10.9861373773513));
#5608=CARTESIAN_POINT('',(0.0114691062182498,2.46092455378925E-15,10.9861373773513));
#5609=CARTESIAN_POINT('Origin',(-26.6060488121491,30.0570908269895,8.98613737735134));
#5610=CARTESIAN_POINT('',(-26.6064009422907,28.0570908269895,10.9861373773513));
#5611=CARTESIAN_POINT('',(-26.6060488121491,28.0570908269895,15.8361373773513));
#5612=CARTESIAN_POINT('',(-26.6064009422907,30.0570908269895,10.9861373773513));
#5613=CARTESIAN_POINT('Origin',(-27.075934518241,30.0570908269895,26.9411392547891));
#5614=CARTESIAN_POINT('',(-31.5209345182411,28.0570908269895,26.9411392547891));
#5615=CARTESIAN_POINT('Origin',(-27.075934518241,28.0570908269895,26.9411392547891));
#5616=CARTESIAN_POINT('',(-31.5209345182411,30.0570908269895,26.9411392547891));
#5617=CARTESIAN_POINT('',(-31.520934518241,30.0570908269895,26.9411392547891));
#5618=CARTESIAN_POINT('Origin',(-27.075934518241,30.0570908269895,26.9411392547891));
#5619=CARTESIAN_POINT('Origin',(21.2986430042118,30.0570908269895,26.4627140227474));
#5620=CARTESIAN_POINT('',(21.2986430042118,30.0570908269895,26.4627140227474));
#5621=CARTESIAN_POINT('',(21.2986430042118,30.0570908269895,27.3527140227474));
#5622=CARTESIAN_POINT('',(21.2986430042118,30.0570908269895,26.4627140227474));
#5623=CARTESIAN_POINT('',(21.2986430042118,28.0570908269895,26.4627140227474));
#5624=CARTESIAN_POINT('',(21.2986430042118,30.0570908269895,26.4627140227474));
#5625=CARTESIAN_POINT('',(21.2986430042118,28.0570908269895,27.3527140227474));
#5626=CARTESIAN_POINT('',(21.2986430042118,28.0570908269895,26.4627140227474));
#5627=CARTESIAN_POINT('',(21.2986430042118,30.0570908269895,27.3527140227474));
#5628=CARTESIAN_POINT('Origin',(17.2986430042118,30.0570908269895,26.4627140227474));
#5629=CARTESIAN_POINT('',(17.2986430042118,30.0570908269895,22.4627140227474));
#5630=CARTESIAN_POINT('Origin',(17.2986430042118,30.0570908269895,26.4627140227474));
#5631=CARTESIAN_POINT('',(17.2986430042118,28.0570908269895,22.4627140227474));
#5632=CARTESIAN_POINT('',(17.2986430042118,30.0570908269895,22.4627140227474));
#5633=CARTESIAN_POINT('Origin',(17.2986430042118,28.0570908269895,26.4627140227474));
#5634=CARTESIAN_POINT('Origin',(13.8686430042118,30.0570908269895,22.4627140227474));
#5635=CARTESIAN_POINT('',(13.8686430042118,30.0570908269895,22.4627140227474));
#5636=CARTESIAN_POINT('',(13.8686430042118,30.0570908269895,22.4627140227474));
#5637=CARTESIAN_POINT('',(13.8686430042118,28.0570908269895,22.4627140227474));
#5638=CARTESIAN_POINT('',(13.8686430042118,30.0570908269895,22.4627140227474));
#5639=CARTESIAN_POINT('',(13.8686430042118,28.0570908269895,22.4627140227474));
#5640=CARTESIAN_POINT('Origin',(13.8686430042118,30.0570908269895,26.4627140227474));
#5641=CARTESIAN_POINT('',(9.86864300421174,30.0570908269895,26.4627140227474));
#5642=CARTESIAN_POINT('Origin',(13.8686430042118,30.0570908269895,26.4627140227474));
#5643=CARTESIAN_POINT('',(9.86864300421174,28.0570908269895,26.4627140227474));
#5644=CARTESIAN_POINT('',(9.86864300421174,30.0570908269895,26.4627140227474));
#5645=CARTESIAN_POINT('Origin',(13.8686430042118,28.0570908269895,26.4627140227474));
#5646=CARTESIAN_POINT('Origin',(9.86864300421174,30.0570908269895,27.3527140227474));
#5647=CARTESIAN_POINT('',(9.86864300421174,30.0570908269895,27.3527140227474));
#5648=CARTESIAN_POINT('',(9.86864300421174,30.0570908269895,27.3527140227474));
#5649=CARTESIAN_POINT('',(9.86864300421174,28.0570908269895,27.3527140227474));
#5650=CARTESIAN_POINT('',(9.86864300421174,30.0570908269895,27.3527140227474));
#5651=CARTESIAN_POINT('',(9.86864300421174,28.0570908269895,27.3527140227474));
#5652=CARTESIAN_POINT('Origin',(13.8686430042118,30.0570908269895,27.3527140227474));
#5653=CARTESIAN_POINT('',(13.8686430042118,30.0570908269895,31.3527140227474));
#5654=CARTESIAN_POINT('Origin',(13.8686430042118,30.0570908269895,27.3527140227474));
#5655=CARTESIAN_POINT('',(13.8686430042118,28.0570908269895,31.3527140227474));
#5656=CARTESIAN_POINT('',(13.8686430042118,30.0570908269895,31.3527140227474));
#5657=CARTESIAN_POINT('Origin',(13.8686430042118,28.0570908269895,27.3527140227474));
#5658=CARTESIAN_POINT('Origin',(17.2986430042118,30.0570908269895,31.3527140227474));
#5659=CARTESIAN_POINT('',(17.2986430042118,30.0570908269895,31.3527140227474));
#5660=CARTESIAN_POINT('',(17.2986430042118,30.0570908269895,31.3527140227474));
#5661=CARTESIAN_POINT('',(17.2986430042118,28.0570908269895,31.3527140227474));
#5662=CARTESIAN_POINT('',(17.2986430042118,30.0570908269895,31.3527140227474));
#5663=CARTESIAN_POINT('',(17.2986430042118,28.0570908269895,31.3527140227474));
#5664=CARTESIAN_POINT('Origin',(17.2986430042118,30.0570908269895,27.3527140227474));
#5665=CARTESIAN_POINT('Origin',(17.2986430042118,30.0570908269895,27.3527140227474));
#5666=CARTESIAN_POINT('Origin',(17.2986430042118,28.0570908269895,27.3527140227474));
#5667=CARTESIAN_POINT('Origin',(-28.773048812149,30.0570908269895,25.8442305588067));
#5668=CARTESIAN_POINT('',(-30.9687372874527,30.0570908269895,19.197505642021));
#5669=CARTESIAN_POINT('',(-35.7730488121491,30.0570908269895,25.8442305588067));
#5670=CARTESIAN_POINT('Origin',(-28.773048812149,30.0570908269895,25.8442305588067));
#5671=CARTESIAN_POINT('',(-30.9687372874527,28.0570908269895,19.197505642021));
#5672=CARTESIAN_POINT('',(-30.9687372874527,30.0570908269895,19.197505642021));
#5673=CARTESIAN_POINT('',(-35.7730488121491,28.0570908269895,25.8442305588067));
#5674=CARTESIAN_POINT('Origin',(-28.773048812149,28.0570908269895,25.8442305588067));
#5675=CARTESIAN_POINT('',(-35.7730488121491,30.0570908269895,25.8442305588067));
#5676=CARTESIAN_POINT('Origin',(-36.5158325318825,30.0570908269895,10.9861373773513));
#5677=CARTESIAN_POINT('Origin',(-36.5158325318825,28.0570908269895,10.9861373773513));
#5678=CARTESIAN_POINT('Origin',(-36.5158325318825,30.0570908269895,10.9861373773513));
#5679=CARTESIAN_POINT('Origin',(19.3037866333901,30.0570908269895,15.0708658676184));
#5680=CARTESIAN_POINT('',(19.3037866333901,30.0570908269895,20.0708658676184));
#5681=CARTESIAN_POINT('Origin',(19.3037866333901,30.0570908269895,15.0708658676184));
#5682=CARTESIAN_POINT('',(19.3037866333901,28.0570908269895,20.0708658676184));
#5683=CARTESIAN_POINT('',(19.3037866333901,30.0570908269895,20.0708658676184));
#5684=CARTESIAN_POINT('Origin',(19.3037866333901,28.0570908269895,15.0708658676184));
#5685=CARTESIAN_POINT('Origin',(19.1869511878509,30.0570908269895,20.0708658676184));
#5686=CARTESIAN_POINT('',(19.1869511878509,30.0570908269895,20.0708658676184));
#5687=CARTESIAN_POINT('',(19.1869511878509,30.0570908269895,20.0708658676184));
#5688=CARTESIAN_POINT('',(19.1869511878509,28.0570908269895,20.0708658676183));
#5689=CARTESIAN_POINT('',(19.1869511878509,30.0570908269895,20.0708658676184));
#5690=CARTESIAN_POINT('',(19.1869511878509,28.0570908269895,20.0708658676184));
#5691=CARTESIAN_POINT('Origin',(19.1869511878509,30.0570908269895,26.0708658676183));
#5692=CARTESIAN_POINT('',(25.1869511878509,30.0570908269895,26.0708658676183));
#5693=CARTESIAN_POINT('Origin',(19.1869511878509,30.0570908269895,26.0708658676183));
#5694=CARTESIAN_POINT('',(25.1869511878509,28.0570908269895,26.0708658676183));
#5695=CARTESIAN_POINT('',(25.1869511878509,30.0570908269895,26.0708658676183));
#5696=CARTESIAN_POINT('Origin',(19.1869511878509,28.0570908269895,26.0708658676183));
#5697=CARTESIAN_POINT('Origin',(25.1869511878509,30.0570908269895,28.3861373773513));
#5698=CARTESIAN_POINT('',(25.1869511878509,30.0570908269895,28.3861373773513));
#5699=CARTESIAN_POINT('',(25.1869511878509,30.0570908269895,34.3861373773513));
#5700=CARTESIAN_POINT('',(25.1869511878509,28.0570908269895,28.3861373773513));
#5701=CARTESIAN_POINT('',(25.1869511878509,30.0570908269895,28.3861373773513));
#5702=CARTESIAN_POINT('',(25.1869511878509,28.0570908269895,34.3861373773513));
#5703=CARTESIAN_POINT('Origin',(19.1869511878509,30.0570908269895,28.3861373773514));
#5704=CARTESIAN_POINT('',(19.1869511878509,30.0570908269895,34.3861373773513));
#5705=CARTESIAN_POINT('Origin',(19.1869511878509,30.0570908269895,28.3861373773514));
#5706=CARTESIAN_POINT('',(19.1869511878509,28.0570908269895,34.3861373773513));
#5707=CARTESIAN_POINT('',(19.1869511878509,30.0570908269895,34.3861373773513));
#5708=CARTESIAN_POINT('Origin',(19.1869511878509,28.0570908269895,28.3861373773513));
#5709=CARTESIAN_POINT('Origin',(-28.773048812149,30.0570908269895,34.3861373773513));
#5710=CARTESIAN_POINT('',(-28.773048812149,30.0570908269895,34.3861373773513));
#5711=CARTESIAN_POINT('',(-35.7730488121491,30.0570908269895,34.3861373773513));
#5712=CARTESIAN_POINT('',(-28.773048812149,28.0570908269895,34.3861373773513));
#5713=CARTESIAN_POINT('',(-28.773048812149,30.0570908269895,34.3861373773513));
#5714=CARTESIAN_POINT('',(-35.7730488121491,28.0570908269895,34.3861373773513));
#5715=CARTESIAN_POINT('Origin',(-28.773048812149,30.0570908269895,27.3861373773513));
#5716=CARTESIAN_POINT('',(-35.7730488121491,30.0570908269895,27.3861373773513));
#5717=CARTESIAN_POINT('Origin',(-28.773048812149,30.0570908269895,27.3861373773513));
#5718=CARTESIAN_POINT('',(-35.7730488121491,28.0570908269895,27.3861373773513));
#5719=CARTESIAN_POINT('',(-35.7730488121491,30.0570908269895,27.3861373773513));
#5720=CARTESIAN_POINT('Origin',(-28.773048812149,28.0570908269895,27.3861373773513));
#5721=CARTESIAN_POINT('Origin',(-35.7730488121491,30.0570908269895,25.8442305588067));
#5722=CARTESIAN_POINT('',(-35.7730488121491,30.0570908269895,25.8442305588067));
#5723=CARTESIAN_POINT('',(-35.7730488121491,28.0570908269895,25.8442305588067));
#5724=CARTESIAN_POINT('Origin',(-5.29304881214906,28.0570908269895,22.6861373773513));
#5725=CARTESIAN_POINT('Origin',(-5.29304881214906,30.0570908269895,22.6861373773513));
#51535=UNCERTAINTY_MEASURE_WITH_UNIT(LENGTH_MEASURE(0.01),#51554,
'DISTANCE_ACCURACY_VALUE',
'Maximum model space distance between geometric entities at asserted c
onnectivities');
#51543=UNCERTAINTY_MEASURE_WITH_UNIT(LENGTH_MEASURE(0.01),#51554,
'DISTANCE_ACCURACY_VALUE',
'Maximum model space distance between geometric entities at asserted c
onnectivities');
#51545=(
GEOMETRIC_REPRESENTATION_CONTEXT(3)
GLOBAL_UNCERTAINTY_ASSIGNED_CONTEXT((#51535))
GLOBAL_UNIT_ASSIGNED_CONTEXT((#51554,#51556,#51557))
REPRESENTATION_CONTEXT('','3D')
);
#51553=(
GEOMETRIC_REPRESENTATION_CONTEXT(3)
GLOBAL_UNCERTAINTY_ASSIGNED_CONTEXT((#51543))
GLOBAL_UNIT_ASSIGNED_CONTEXT((#51554,#51556,#51557))
REPRESENTATION_CONTEXT('','3D')
);
#51554=(
LENGTH_UNIT()
NAMED_UNIT(*)
SI_UNIT(.MILLI.,.METRE.)
);
#51556=(
NAMED_UNIT(*)
PLANE_ANGLE_UNIT()
SI_UNIT($,.RADIAN.)
);
#51557=(
NAMED_UNIT(*)
SI_UNIT($,.STERADIAN.)
SOLID_ANGLE_UNIT()
);
#51559=SHAPE_DEFINITION_REPRESENTATION(#51568,#51585);
#51568=PRODUCT_DEFINITION_SHAPE('',$,#51595);
#51585=SHAPE_REPRESENTATION('',(#4358),#51545);
#51593=PRODUCT_DEFINITION_CONTEXT('part definition',#51622,'design');
#51595=PRODUCT_DEFINITION('Clamp_01','Clamp_01',#51604,#51593);
#51604=PRODUCT_DEFINITION_FORMATION('',$,#51625);
#51622=APPLICATION_CONTEXT(
'Core Data for Automotive Mechanical Design Process');
#51623=PRODUCT_CONTEXT('part definition',#51622,'mechanical');
#51625=PRODUCT('Clamp_01','Clamp_01',$,(#51623));
#51634=PRESENTATION_STYLE_ASSIGNMENT((#51637));
#51637=SURFACE_STYLE_USAGE(.BOTH.,#51640);
#51640=SURFACE_SIDE_STYLE('',(#51643));
#51643=SURFACE_STYLE_FILL_AREA(#51646);
#51646=FILL_AREA_STYLE('Opaque(203,203,203)',(#51649));
#51649=FILL_AREA_STYLE_COLOUR('Opaque(203,203,203)',#51652);
#51652=COLOUR_RGB('Opaque(203,203,203)', 0.09019608, 0.27058824, 0.51372549);
ENDSEC;
END-ISO-10303-21;
